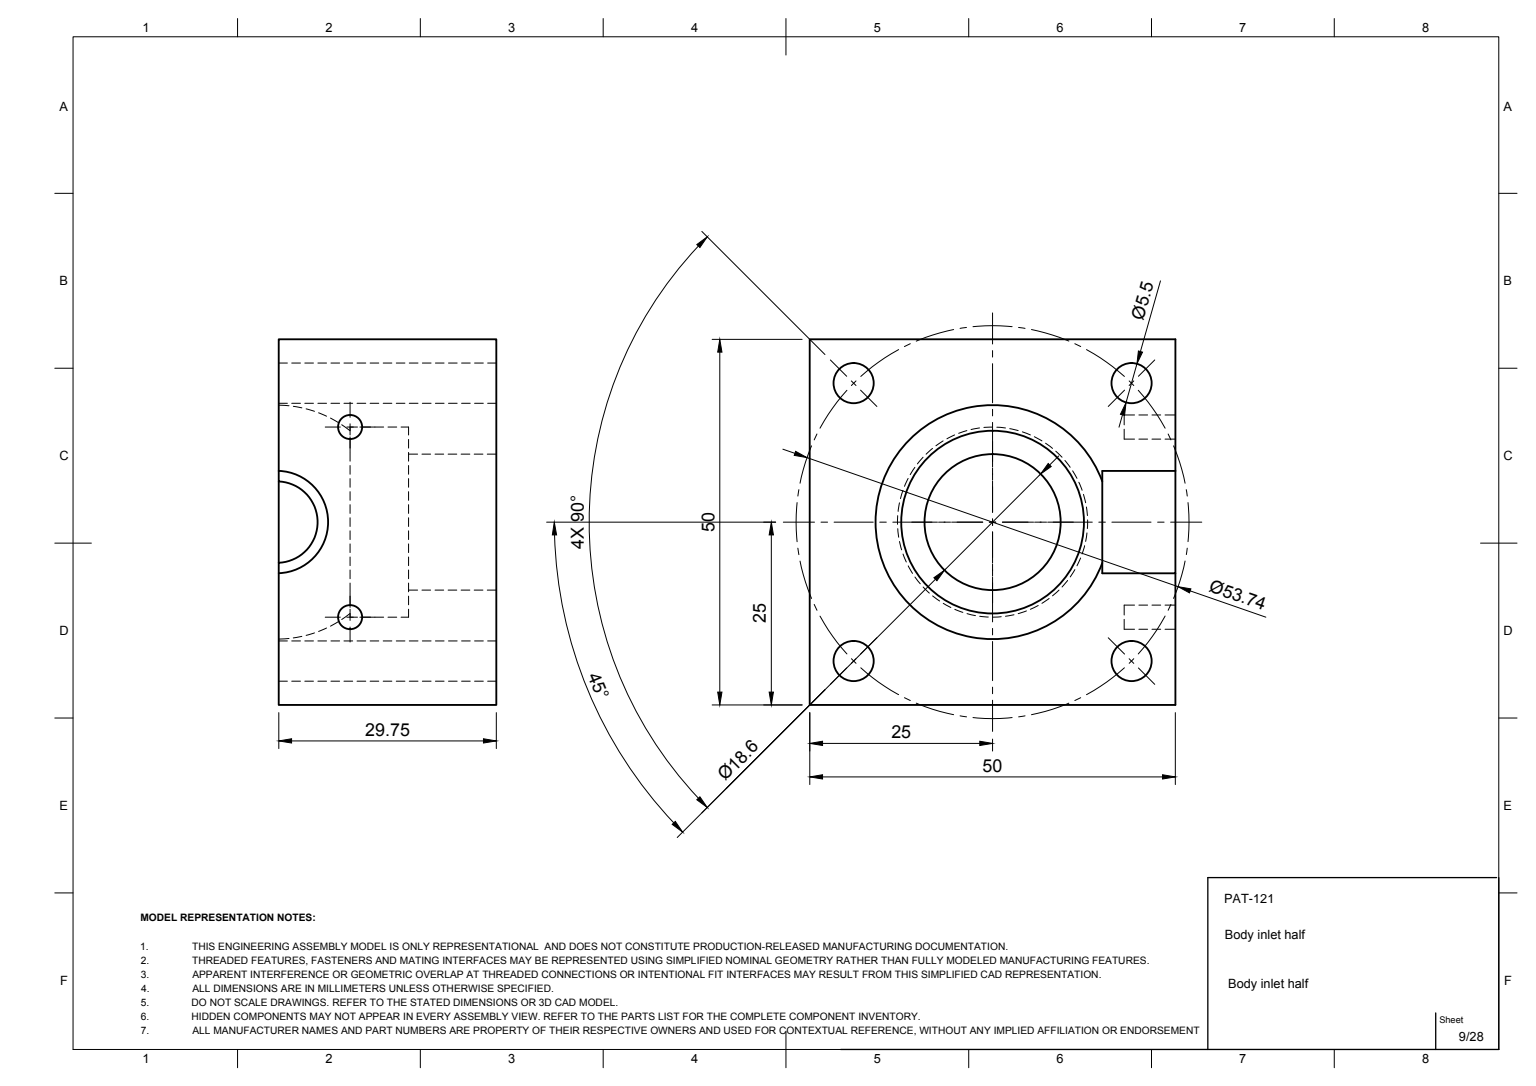
ISO-10303-21;
HEADER;
/* Generated by software containing ST-Developer
 * from STEP Tools, Inc. (www.steptools.com) 
 */

FILE_DESCRIPTION(
/* description */ ('Wall-mounted air drop station'),
/* implementation_level */ '2;1');

FILE_NAME(
/* name */ 'Body inlet half.step',
/* time_stamp */ '2026-10-28T22:16:19-07:00',
/* author */ (''),
/* organization */ (''),
/* preprocessor_version */ 'ST-DEVELOPER v20.2',
/* originating_system */ 'Autodesk Translation Framework v15.17.0.0',
/* authorisation */ '');

FILE_SCHEMA (('AUTOMOTIVE_DESIGN { 1 0 10303 214 3 1 1 }'));
ENDSEC;

DATA;
#10=MECHANICAL_DESIGN_GEOMETRIC_PRESENTATION_REPRESENTATION('',(#349),#10517);
#258=SPHERICAL_SURFACE('',#6417,1.6);
#291=SHAPE_REPRESENTATION_RELATIONSHIP('SRR','None',#10648,#320);
#320=ADVANCED_BREP_SHAPE_REPRESENTATION('',(#378),#10492);
#349=STYLED_ITEM('',(#10853),#378);
#378=MANIFOLD_SOLID_BREP('Body1',#5888);
#435=FACE_BOUND('',#1240,.T.);
#436=FACE_BOUND('',#1241,.T.);
#437=FACE_BOUND('',#1245,.T.);
#438=FACE_BOUND('',#1247,.T.);
#439=FACE_BOUND('',#1249,.T.);
#440=FACE_BOUND('',#1251,.T.);
#441=FACE_BOUND('',#1252,.T.);
#442=FACE_BOUND('',#1253,.T.);
#443=FACE_BOUND('',#1254,.T.);
#444=FACE_BOUND('',#1257,.T.);
#445=FACE_BOUND('',#1258,.T.);
#446=FACE_BOUND('',#1259,.T.);
#447=FACE_BOUND('',#1260,.T.);
#448=FACE_BOUND('',#1261,.T.);
#580=PLANE('',#6385);
#581=PLANE('',#6389);
#582=PLANE('',#6405);
#583=PLANE('',#6407);
#584=PLANE('',#6414);
#585=PLANE('',#6416);
#586=PLANE('',#6419);
#587=PLANE('',#6420);
#588=PLANE('',#6421);
#589=PLANE('',#6422);
#590=PLANE('',#6423);
#838=FACE_OUTER_BOUND('',#1229,.T.);
#839=FACE_OUTER_BOUND('',#1230,.T.);
#840=FACE_OUTER_BOUND('',#1231,.T.);
#841=FACE_OUTER_BOUND('',#1232,.T.);
#842=FACE_OUTER_BOUND('',#1233,.T.);
#843=FACE_OUTER_BOUND('',#1234,.T.);
#844=FACE_OUTER_BOUND('',#1235,.T.);
#845=FACE_OUTER_BOUND('',#1236,.T.);
#846=FACE_OUTER_BOUND('',#1237,.T.);
#847=FACE_OUTER_BOUND('',#1238,.T.);
#848=FACE_OUTER_BOUND('',#1239,.T.);
#849=FACE_OUTER_BOUND('',#1242,.T.);
#850=FACE_OUTER_BOUND('',#1243,.T.);
#851=FACE_OUTER_BOUND('',#1244,.T.);
#852=FACE_OUTER_BOUND('',#1246,.T.);
#853=FACE_OUTER_BOUND('',#1248,.T.);
#854=FACE_OUTER_BOUND('',#1250,.T.);
#855=FACE_OUTER_BOUND('',#1255,.T.);
#856=FACE_OUTER_BOUND('',#1256,.T.);
#857=FACE_OUTER_BOUND('',#1262,.T.);
#858=FACE_OUTER_BOUND('',#1263,.T.);
#1229=EDGE_LOOP('',(#4323,#4324,#4325,#4326));
#1230=EDGE_LOOP('',(#4327));
#1231=EDGE_LOOP('',(#4328,#4329,#4330,#4331));
#1232=EDGE_LOOP('',(#4332));
#1233=EDGE_LOOP('',(#4333,#4334,#4335,#4336));
#1234=EDGE_LOOP('',(#4337,#4338,#4339,#4340));
#1235=EDGE_LOOP('',(#4341,#4342,#4343,#4344));
#1236=EDGE_LOOP('',(#4345,#4346,#4347,#4348));
#1237=EDGE_LOOP('',(#4349,#4350,#4351,#4352));
#1238=EDGE_LOOP('',(#4353,#4354,#4355,#4356));
#1239=EDGE_LOOP('',(#4357,#4358,#4359,#4360,#4361,#4362));
#1240=EDGE_LOOP('',(#4363));
#1241=EDGE_LOOP('',(#4364));
#1242=EDGE_LOOP('',(#4365,#4366,#4367,#4368));
#1243=EDGE_LOOP('',(#4369,#4370,#4371,#4372));
#1244=EDGE_LOOP('',(#4373));
#1245=EDGE_LOOP('',(#4374));
#1246=EDGE_LOOP('',(#4375));
#1247=EDGE_LOOP('',(#4376));
#1248=EDGE_LOOP('',(#4377,#4378));
#1249=EDGE_LOOP('',(#4379));
#1250=EDGE_LOOP('',(#4380,#4381,#4382,#4383,#4384,#4385,#4386,#4387,#4388,
#4389));
#1251=EDGE_LOOP('',(#4390));
#1252=EDGE_LOOP('',(#4391));
#1253=EDGE_LOOP('',(#4392));
#1254=EDGE_LOOP('',(#4393));
#1255=EDGE_LOOP('',(#4394,#4395,#4396,#4397));
#1256=EDGE_LOOP('',(#4398,#4399,#4400,#4401));
#1257=EDGE_LOOP('',(#4402));
#1258=EDGE_LOOP('',(#4403));
#1259=EDGE_LOOP('',(#4404));
#1260=EDGE_LOOP('',(#4405));
#1261=EDGE_LOOP('',(#4406));
#1262=EDGE_LOOP('',(#4407,#4408,#4409,#4410));
#1263=EDGE_LOOP('',(#4411,#4412,#4413,#4414));
#1711=LINE('',#9152,#2175);
#1712=LINE('',#9159,#2176);
#1713=LINE('',#9166,#2177);
#1714=LINE('',#9172,#2178);
#1715=LINE('',#9178,#2179);
#1716=LINE('',#9184,#2180);
#1717=LINE('',#9189,#2181);
#1718=LINE('',#9193,#2182);
#1719=LINE('',#9197,#2183);
#1720=LINE('',#9200,#2184);
#1721=LINE('',#9203,#2185);
#1722=LINE('',#9205,#2186);
#1723=LINE('',#9207,#2187);
#1724=LINE('',#9209,#2188);
#1725=LINE('',#9210,#2189);
#1726=LINE('',#9215,#2190);
#1727=LINE('',#9221,#2191);
#1728=LINE('',#9231,#2192);
#1729=LINE('',#9233,#2193);
#1730=LINE('',#9234,#2194);
#1731=LINE('',#9237,#2195);
#1732=LINE('',#9238,#2196);
#1733=LINE('',#9241,#2197);
#1734=LINE('',#9242,#2198);
#1735=LINE('',#9244,#2199);
#2175=VECTOR('',#7341,0.165);
#2176=VECTOR('',#7350,0.165);
#2177=VECTOR('',#7359,0.275);
#2178=VECTOR('',#7366,0.275);
#2179=VECTOR('',#7373,0.275);
#2180=VECTOR('',#7380,0.275);
#2181=VECTOR('',#7385,1.);
#2182=VECTOR('',#7388,1.);
#2183=VECTOR('',#7393,1.);
#2184=VECTOR('',#7396,1.);
#2185=VECTOR('',#7399,1.);
#2186=VECTOR('',#7400,1.);
#2187=VECTOR('',#7401,1.);
#2188=VECTOR('',#7402,1.);
#2189=VECTOR('',#7403,1.);
#2190=VECTOR('',#7408,0.93);
#2191=VECTOR('',#7415,1.3);
#2192=VECTOR('',#7430,1.);
#2193=VECTOR('',#7431,1.);
#2194=VECTOR('',#7432,1.);
#2195=VECTOR('',#7435,1.);
#2196=VECTOR('',#7436,1.);
#2197=VECTOR('',#7439,1.);
#2198=VECTOR('',#7440,1.);
#2199=VECTOR('',#7443,1.);
#2576=CIRCLE('',#6383,0.165);
#2577=CIRCLE('',#6384,0.165);
#2578=CIRCLE('',#6387,0.165);
#2579=CIRCLE('',#6388,0.165);
#2580=CIRCLE('',#6391,0.275);
#2581=CIRCLE('',#6392,0.275);
#2582=CIRCLE('',#6394,0.275);
#2583=CIRCLE('',#6395,0.275);
#2584=CIRCLE('',#6397,0.275);
#2585=CIRCLE('',#6398,0.275);
#2586=CIRCLE('',#6400,0.275);
#2587=CIRCLE('',#6401,0.275);
#2588=CIRCLE('',#6403,0.7);
#2589=CIRCLE('',#6404,0.7);
#2590=CIRCLE('',#6406,0.556776436283003);
#2591=CIRCLE('',#6409,0.93);
#2592=CIRCLE('',#6410,0.93);
#2593=CIRCLE('',#6412,1.3);
#2594=CIRCLE('',#6413,1.3);
#2595=CIRCLE('',#6415,1.24899959967968);
#2596=CIRCLE('',#6418,1.59980467557762);
#2881=VERTEX_POINT('',#9149);
#2882=VERTEX_POINT('',#9151);
#2883=VERTEX_POINT('',#9156);
#2884=VERTEX_POINT('',#9158);
#2885=VERTEX_POINT('',#9163);
#2886=VERTEX_POINT('',#9165);
#2887=VERTEX_POINT('',#9169);
#2888=VERTEX_POINT('',#9171);
#2889=VERTEX_POINT('',#9175);
#2890=VERTEX_POINT('',#9177);
#2891=VERTEX_POINT('',#9181);
#2892=VERTEX_POINT('',#9183);
#2893=VERTEX_POINT('',#9187);
#2894=VERTEX_POINT('',#9188);
#2895=VERTEX_POINT('',#9190);
#2896=VERTEX_POINT('',#9192);
#2897=VERTEX_POINT('',#9196);
#2898=VERTEX_POINT('',#9198);
#2899=VERTEX_POINT('',#9202);
#2900=VERTEX_POINT('',#9204);
#2901=VERTEX_POINT('',#9206);
#2902=VERTEX_POINT('',#9208);
#2903=VERTEX_POINT('',#9212);
#2904=VERTEX_POINT('',#9214);
#2905=VERTEX_POINT('',#9218);
#2906=VERTEX_POINT('',#9220);
#2907=VERTEX_POINT('',#9224);
#2908=VERTEX_POINT('',#9230);
#2909=VERTEX_POINT('',#9232);
#2910=VERTEX_POINT('',#9236);
#2911=VERTEX_POINT('',#9240);
#3419=EDGE_CURVE('',#2881,#2881,#2576,.T.);
#3420=EDGE_CURVE('',#2881,#2882,#1711,.T.);
#3421=EDGE_CURVE('',#2882,#2882,#2577,.T.);
#3422=EDGE_CURVE('',#2883,#2883,#2578,.T.);
#3423=EDGE_CURVE('',#2883,#2884,#1712,.T.);
#3424=EDGE_CURVE('',#2884,#2884,#2579,.T.);
#3425=EDGE_CURVE('',#2885,#2885,#2580,.T.);
#3426=EDGE_CURVE('',#2885,#2886,#1713,.T.);
#3427=EDGE_CURVE('',#2886,#2886,#2581,.T.);
#3428=EDGE_CURVE('',#2887,#2887,#2582,.T.);
#3429=EDGE_CURVE('',#2887,#2888,#1714,.T.);
#3430=EDGE_CURVE('',#2888,#2888,#2583,.T.);
#3431=EDGE_CURVE('',#2889,#2889,#2584,.T.);
#3432=EDGE_CURVE('',#2889,#2890,#1715,.T.);
#3433=EDGE_CURVE('',#2890,#2890,#2585,.T.);
#3434=EDGE_CURVE('',#2891,#2891,#2586,.T.);
#3435=EDGE_CURVE('',#2891,#2892,#1716,.T.);
#3436=EDGE_CURVE('',#2892,#2892,#2587,.T.);
#3437=EDGE_CURVE('',#2893,#2894,#1717,.T.);
#3438=EDGE_CURVE('',#2895,#2893,#2588,.T.);
#3439=EDGE_CURVE('',#2896,#2895,#1718,.T.);
#3440=EDGE_CURVE('',#2894,#2896,#2589,.T.);
#3441=EDGE_CURVE('',#2897,#2893,#1719,.T.);
#3442=EDGE_CURVE('',#2898,#2897,#2590,.T.);
#3443=EDGE_CURVE('',#2895,#2898,#1720,.T.);
#3444=EDGE_CURVE('',#2896,#2899,#1721,.T.);
#3445=EDGE_CURVE('',#2899,#2900,#1722,.T.);
#3446=EDGE_CURVE('',#2900,#2901,#1723,.T.);
#3447=EDGE_CURVE('',#2901,#2902,#1724,.T.);
#3448=EDGE_CURVE('',#2902,#2894,#1725,.T.);
#3449=EDGE_CURVE('',#2903,#2903,#2591,.T.);
#3450=EDGE_CURVE('',#2903,#2904,#1726,.T.);
#3451=EDGE_CURVE('',#2904,#2904,#2592,.T.);
#3452=EDGE_CURVE('',#2905,#2905,#2593,.T.);
#3453=EDGE_CURVE('',#2905,#2906,#1727,.T.);
#3454=EDGE_CURVE('',#2906,#2906,#2594,.T.);
#3455=EDGE_CURVE('',#2907,#2907,#2595,.T.);
#3456=EDGE_CURVE('',#2898,#2897,#2596,.T.);
#3457=EDGE_CURVE('',#2908,#2902,#1728,.T.);
#3458=EDGE_CURVE('',#2908,#2909,#1729,.T.);
#3459=EDGE_CURVE('',#2909,#2899,#1730,.T.);
#3460=EDGE_CURVE('',#2910,#2908,#1731,.T.);
#3461=EDGE_CURVE('',#2910,#2901,#1732,.T.);
#3462=EDGE_CURVE('',#2911,#2910,#1733,.T.);
#3463=EDGE_CURVE('',#2911,#2900,#1734,.T.);
#3464=EDGE_CURVE('',#2909,#2911,#1735,.T.);
#4323=ORIENTED_EDGE('',*,*,#3419,.F.);
#4324=ORIENTED_EDGE('',*,*,#3420,.T.);
#4325=ORIENTED_EDGE('',*,*,#3421,.F.);
#4326=ORIENTED_EDGE('',*,*,#3420,.F.);
#4327=ORIENTED_EDGE('',*,*,#3419,.T.);
#4328=ORIENTED_EDGE('',*,*,#3422,.F.);
#4329=ORIENTED_EDGE('',*,*,#3423,.T.);
#4330=ORIENTED_EDGE('',*,*,#3424,.F.);
#4331=ORIENTED_EDGE('',*,*,#3423,.F.);
#4332=ORIENTED_EDGE('',*,*,#3422,.T.);
#4333=ORIENTED_EDGE('',*,*,#3425,.F.);
#4334=ORIENTED_EDGE('',*,*,#3426,.T.);
#4335=ORIENTED_EDGE('',*,*,#3427,.F.);
#4336=ORIENTED_EDGE('',*,*,#3426,.F.);
#4337=ORIENTED_EDGE('',*,*,#3428,.F.);
#4338=ORIENTED_EDGE('',*,*,#3429,.T.);
#4339=ORIENTED_EDGE('',*,*,#3430,.F.);
#4340=ORIENTED_EDGE('',*,*,#3429,.F.);
#4341=ORIENTED_EDGE('',*,*,#3431,.F.);
#4342=ORIENTED_EDGE('',*,*,#3432,.T.);
#4343=ORIENTED_EDGE('',*,*,#3433,.F.);
#4344=ORIENTED_EDGE('',*,*,#3432,.F.);
#4345=ORIENTED_EDGE('',*,*,#3434,.F.);
#4346=ORIENTED_EDGE('',*,*,#3435,.T.);
#4347=ORIENTED_EDGE('',*,*,#3436,.F.);
#4348=ORIENTED_EDGE('',*,*,#3435,.F.);
#4349=ORIENTED_EDGE('',*,*,#3437,.F.);
#4350=ORIENTED_EDGE('',*,*,#3438,.F.);
#4351=ORIENTED_EDGE('',*,*,#3439,.F.);
#4352=ORIENTED_EDGE('',*,*,#3440,.F.);
#4353=ORIENTED_EDGE('',*,*,#3441,.F.);
#4354=ORIENTED_EDGE('',*,*,#3442,.F.);
#4355=ORIENTED_EDGE('',*,*,#3443,.F.);
#4356=ORIENTED_EDGE('',*,*,#3438,.T.);
#4357=ORIENTED_EDGE('',*,*,#3440,.T.);
#4358=ORIENTED_EDGE('',*,*,#3444,.T.);
#4359=ORIENTED_EDGE('',*,*,#3445,.T.);
#4360=ORIENTED_EDGE('',*,*,#3446,.T.);
#4361=ORIENTED_EDGE('',*,*,#3447,.T.);
#4362=ORIENTED_EDGE('',*,*,#3448,.T.);
#4363=ORIENTED_EDGE('',*,*,#3421,.T.);
#4364=ORIENTED_EDGE('',*,*,#3424,.T.);
#4365=ORIENTED_EDGE('',*,*,#3449,.F.);
#4366=ORIENTED_EDGE('',*,*,#3450,.T.);
#4367=ORIENTED_EDGE('',*,*,#3451,.F.);
#4368=ORIENTED_EDGE('',*,*,#3450,.F.);
#4369=ORIENTED_EDGE('',*,*,#3452,.F.);
#4370=ORIENTED_EDGE('',*,*,#3453,.T.);
#4371=ORIENTED_EDGE('',*,*,#3454,.T.);
#4372=ORIENTED_EDGE('',*,*,#3453,.F.);
#4373=ORIENTED_EDGE('',*,*,#3454,.F.);
#4374=ORIENTED_EDGE('',*,*,#3455,.F.);
#4375=ORIENTED_EDGE('',*,*,#3452,.T.);
#4376=ORIENTED_EDGE('',*,*,#3451,.T.);
#4377=ORIENTED_EDGE('',*,*,#3442,.T.);
#4378=ORIENTED_EDGE('',*,*,#3456,.F.);
#4379=ORIENTED_EDGE('',*,*,#3455,.T.);
#4380=ORIENTED_EDGE('',*,*,#3437,.T.);
#4381=ORIENTED_EDGE('',*,*,#3448,.F.);
#4382=ORIENTED_EDGE('',*,*,#3457,.F.);
#4383=ORIENTED_EDGE('',*,*,#3458,.T.);
#4384=ORIENTED_EDGE('',*,*,#3459,.T.);
#4385=ORIENTED_EDGE('',*,*,#3444,.F.);
#4386=ORIENTED_EDGE('',*,*,#3439,.T.);
#4387=ORIENTED_EDGE('',*,*,#3443,.T.);
#4388=ORIENTED_EDGE('',*,*,#3456,.T.);
#4389=ORIENTED_EDGE('',*,*,#3441,.T.);
#4390=ORIENTED_EDGE('',*,*,#3427,.T.);
#4391=ORIENTED_EDGE('',*,*,#3430,.T.);
#4392=ORIENTED_EDGE('',*,*,#3433,.T.);
#4393=ORIENTED_EDGE('',*,*,#3436,.T.);
#4394=ORIENTED_EDGE('',*,*,#3460,.T.);
#4395=ORIENTED_EDGE('',*,*,#3457,.T.);
#4396=ORIENTED_EDGE('',*,*,#3447,.F.);
#4397=ORIENTED_EDGE('',*,*,#3461,.F.);
#4398=ORIENTED_EDGE('',*,*,#3462,.T.);
#4399=ORIENTED_EDGE('',*,*,#3461,.T.);
#4400=ORIENTED_EDGE('',*,*,#3446,.F.);
#4401=ORIENTED_EDGE('',*,*,#3463,.F.);
#4402=ORIENTED_EDGE('',*,*,#3449,.T.);
#4403=ORIENTED_EDGE('',*,*,#3434,.T.);
#4404=ORIENTED_EDGE('',*,*,#3431,.T.);
#4405=ORIENTED_EDGE('',*,*,#3428,.T.);
#4406=ORIENTED_EDGE('',*,*,#3425,.T.);
#4407=ORIENTED_EDGE('',*,*,#3464,.T.);
#4408=ORIENTED_EDGE('',*,*,#3463,.T.);
#4409=ORIENTED_EDGE('',*,*,#3445,.F.);
#4410=ORIENTED_EDGE('',*,*,#3459,.F.);
#4411=ORIENTED_EDGE('',*,*,#3464,.F.);
#4412=ORIENTED_EDGE('',*,*,#3458,.F.);
#4413=ORIENTED_EDGE('',*,*,#3460,.F.);
#4414=ORIENTED_EDGE('',*,*,#3462,.F.);
#5457=CYLINDRICAL_SURFACE('',#6382,0.165);
#5458=CYLINDRICAL_SURFACE('',#6386,0.165);
#5459=CYLINDRICAL_SURFACE('',#6390,0.275);
#5460=CYLINDRICAL_SURFACE('',#6393,0.275);
#5461=CYLINDRICAL_SURFACE('',#6396,0.275);
#5462=CYLINDRICAL_SURFACE('',#6399,0.275);
#5463=CYLINDRICAL_SURFACE('',#6402,0.7);
#5464=CYLINDRICAL_SURFACE('',#6408,0.93);
#5465=CYLINDRICAL_SURFACE('',#6411,1.3);
#5611=ADVANCED_FACE('',(#838),#5457,.F.);
#5612=ADVANCED_FACE('',(#839),#580,.T.);
#5613=ADVANCED_FACE('',(#840),#5458,.F.);
#5614=ADVANCED_FACE('',(#841),#581,.T.);
#5615=ADVANCED_FACE('',(#842),#5459,.F.);
#5616=ADVANCED_FACE('',(#843),#5460,.F.);
#5617=ADVANCED_FACE('',(#844),#5461,.F.);
#5618=ADVANCED_FACE('',(#845),#5462,.F.);
#5619=ADVANCED_FACE('',(#846),#5463,.F.);
#5620=ADVANCED_FACE('',(#847),#582,.T.);
#5621=ADVANCED_FACE('',(#848,#435,#436),#583,.T.);
#5622=ADVANCED_FACE('',(#849),#5464,.F.);
#5623=ADVANCED_FACE('',(#850),#5465,.F.);
#5624=ADVANCED_FACE('',(#851,#437),#584,.F.);
#5625=ADVANCED_FACE('',(#852,#438),#585,.T.);
#5626=ADVANCED_FACE('',(#853,#439),#258,.F.);
#5627=ADVANCED_FACE('',(#854,#440,#441,#442,#443),#586,.T.);
#5628=ADVANCED_FACE('',(#855),#587,.T.);
#5629=ADVANCED_FACE('',(#856,#444,#445,#446,#447,#448),#588,.T.);
#5630=ADVANCED_FACE('',(#857),#589,.T.);
#5631=ADVANCED_FACE('',(#858),#590,.F.);
#5888=CLOSED_SHELL('',(#5611,#5612,#5613,#5614,#5615,#5616,#5617,#5618,
#5619,#5620,#5621,#5622,#5623,#5624,#5625,#5626,#5627,#5628,#5629,#5630,
#5631));
#6381=AXIS2_PLACEMENT_3D('',#9147,#7335,#7336);
#6382=AXIS2_PLACEMENT_3D('',#9148,#7337,#7338);
#6383=AXIS2_PLACEMENT_3D('',#9150,#7339,#7340);
#6384=AXIS2_PLACEMENT_3D('',#9153,#7342,#7343);
#6385=AXIS2_PLACEMENT_3D('',#9154,#7344,#7345);
#6386=AXIS2_PLACEMENT_3D('',#9155,#7346,#7347);
#6387=AXIS2_PLACEMENT_3D('',#9157,#7348,#7349);
#6388=AXIS2_PLACEMENT_3D('',#9160,#7351,#7352);
#6389=AXIS2_PLACEMENT_3D('',#9161,#7353,#7354);
#6390=AXIS2_PLACEMENT_3D('',#9162,#7355,#7356);
#6391=AXIS2_PLACEMENT_3D('',#9164,#7357,#7358);
#6392=AXIS2_PLACEMENT_3D('',#9167,#7360,#7361);
#6393=AXIS2_PLACEMENT_3D('',#9168,#7362,#7363);
#6394=AXIS2_PLACEMENT_3D('',#9170,#7364,#7365);
#6395=AXIS2_PLACEMENT_3D('',#9173,#7367,#7368);
#6396=AXIS2_PLACEMENT_3D('',#9174,#7369,#7370);
#6397=AXIS2_PLACEMENT_3D('',#9176,#7371,#7372);
#6398=AXIS2_PLACEMENT_3D('',#9179,#7374,#7375);
#6399=AXIS2_PLACEMENT_3D('',#9180,#7376,#7377);
#6400=AXIS2_PLACEMENT_3D('',#9182,#7378,#7379);
#6401=AXIS2_PLACEMENT_3D('',#9185,#7381,#7382);
#6402=AXIS2_PLACEMENT_3D('',#9186,#7383,#7384);
#6403=AXIS2_PLACEMENT_3D('',#9191,#7386,#7387);
#6404=AXIS2_PLACEMENT_3D('',#9194,#7389,#7390);
#6405=AXIS2_PLACEMENT_3D('',#9195,#7391,#7392);
#6406=AXIS2_PLACEMENT_3D('',#9199,#7394,#7395);
#6407=AXIS2_PLACEMENT_3D('',#9201,#7397,#7398);
#6408=AXIS2_PLACEMENT_3D('',#9211,#7404,#7405);
#6409=AXIS2_PLACEMENT_3D('',#9213,#7406,#7407);
#6410=AXIS2_PLACEMENT_3D('',#9216,#7409,#7410);
#6411=AXIS2_PLACEMENT_3D('',#9217,#7411,#7412);
#6412=AXIS2_PLACEMENT_3D('',#9219,#7413,#7414);
#6413=AXIS2_PLACEMENT_3D('',#9222,#7416,#7417);
#6414=AXIS2_PLACEMENT_3D('',#9223,#7418,#7419);
#6415=AXIS2_PLACEMENT_3D('',#9225,#7420,#7421);
#6416=AXIS2_PLACEMENT_3D('',#9226,#7422,#7423);
#6417=AXIS2_PLACEMENT_3D('',#9227,#7424,#7425);
#6418=AXIS2_PLACEMENT_3D('',#9228,#7426,#7427);
#6419=AXIS2_PLACEMENT_3D('',#9229,#7428,#7429);
#6420=AXIS2_PLACEMENT_3D('',#9235,#7433,#7434);
#6421=AXIS2_PLACEMENT_3D('',#9239,#7437,#7438);
#6422=AXIS2_PLACEMENT_3D('',#9243,#7441,#7442);
#6423=AXIS2_PLACEMENT_3D('',#9245,#7444,#7445);
#7335=DIRECTION('axis',(0.,0.,1.));
#7336=DIRECTION('refdir',(1.,0.,0.));
#7337=DIRECTION('center_axis',(0.,0.,1.));
#7338=DIRECTION('ref_axis',(1.,0.,0.));
#7339=DIRECTION('center_axis',(0.,0.,1.));
#7340=DIRECTION('ref_axis',(1.,0.,0.));
#7341=DIRECTION('',(0.,0.,1.));
#7342=DIRECTION('center_axis',(0.,0.,-1.));
#7343=DIRECTION('ref_axis',(1.,0.,0.));
#7344=DIRECTION('center_axis',(0.,0.,1.));
#7345=DIRECTION('ref_axis',(1.,0.,0.));
#7346=DIRECTION('center_axis',(0.,0.,1.));
#7347=DIRECTION('ref_axis',(1.,0.,0.));
#7348=DIRECTION('center_axis',(0.,0.,1.));
#7349=DIRECTION('ref_axis',(1.,0.,0.));
#7350=DIRECTION('',(0.,0.,1.));
#7351=DIRECTION('center_axis',(0.,0.,-1.));
#7352=DIRECTION('ref_axis',(1.,0.,0.));
#7353=DIRECTION('center_axis',(0.,0.,1.));
#7354=DIRECTION('ref_axis',(1.,0.,0.));
#7355=DIRECTION('center_axis',(0.,1.,0.));
#7356=DIRECTION('ref_axis',(1.,0.,0.));
#7357=DIRECTION('center_axis',(0.,1.,0.));
#7358=DIRECTION('ref_axis',(1.,0.,0.));
#7359=DIRECTION('',(0.,1.,0.));
#7360=DIRECTION('center_axis',(0.,-1.,0.));
#7361=DIRECTION('ref_axis',(1.,0.,0.));
#7362=DIRECTION('center_axis',(0.,1.,0.));
#7363=DIRECTION('ref_axis',(1.,0.,0.));
#7364=DIRECTION('center_axis',(0.,1.,0.));
#7365=DIRECTION('ref_axis',(1.,0.,0.));
#7366=DIRECTION('',(0.,1.,0.));
#7367=DIRECTION('center_axis',(0.,-1.,0.));
#7368=DIRECTION('ref_axis',(1.,0.,0.));
#7369=DIRECTION('center_axis',(0.,1.,0.));
#7370=DIRECTION('ref_axis',(1.,0.,0.));
#7371=DIRECTION('center_axis',(0.,1.,0.));
#7372=DIRECTION('ref_axis',(1.,0.,0.));
#7373=DIRECTION('',(0.,1.,0.));
#7374=DIRECTION('center_axis',(0.,-1.,0.));
#7375=DIRECTION('ref_axis',(1.,0.,0.));
#7376=DIRECTION('center_axis',(0.,1.,0.));
#7377=DIRECTION('ref_axis',(1.,0.,0.));
#7378=DIRECTION('center_axis',(0.,1.,0.));
#7379=DIRECTION('ref_axis',(1.,0.,0.));
#7380=DIRECTION('',(0.,1.,0.));
#7381=DIRECTION('center_axis',(0.,-1.,0.));
#7382=DIRECTION('ref_axis',(1.,0.,0.));
#7383=DIRECTION('center_axis',(0.,0.,1.));
#7384=DIRECTION('ref_axis',(1.,0.,0.));
#7385=DIRECTION('',(0.,0.,1.));
#7386=DIRECTION('center_axis',(0.,0.,1.));
#7387=DIRECTION('ref_axis',(1.,0.,0.));
#7388=DIRECTION('',(0.,0.,-1.));
#7389=DIRECTION('center_axis',(0.,0.,-1.));
#7390=DIRECTION('ref_axis',(1.,0.,0.));
#7391=DIRECTION('center_axis',(0.,0.,1.));
#7392=DIRECTION('ref_axis',(1.,0.,0.));
#7393=DIRECTION('',(1.,0.,0.));
#7394=DIRECTION('center_axis',(0.,0.,1.));
#7395=DIRECTION('ref_axis',(0.,-1.,0.));
#7396=DIRECTION('',(1.,0.,0.));
#7397=DIRECTION('center_axis',(0.,0.,1.));
#7398=DIRECTION('ref_axis',(1.,0.,0.));
#7399=DIRECTION('',(-1.,0.,0.));
#7400=DIRECTION('',(0.,-1.,0.));
#7401=DIRECTION('',(1.,0.,0.));
#7402=DIRECTION('',(0.,1.,0.));
#7403=DIRECTION('',(-1.,0.,0.));
#7404=DIRECTION('center_axis',(0.,1.,0.));
#7405=DIRECTION('ref_axis',(1.,0.,0.));
#7406=DIRECTION('center_axis',(0.,1.,0.));
#7407=DIRECTION('ref_axis',(1.,0.,0.));
#7408=DIRECTION('',(0.,1.,0.));
#7409=DIRECTION('center_axis',(0.,-1.,0.));
#7410=DIRECTION('ref_axis',(1.,0.,0.));
#7411=DIRECTION('center_axis',(0.,1.,0.));
#7412=DIRECTION('ref_axis',(1.,0.,0.));
#7413=DIRECTION('center_axis',(0.,1.,0.));
#7414=DIRECTION('ref_axis',(1.,0.,0.));
#7415=DIRECTION('',(0.,1.,0.));
#7416=DIRECTION('center_axis',(0.,1.,0.));
#7417=DIRECTION('ref_axis',(1.,0.,0.));
#7418=DIRECTION('center_axis',(0.,1.,0.));
#7419=DIRECTION('ref_axis',(1.,0.,0.));
#7420=DIRECTION('center_axis',(0.,-1.,0.));
#7421=DIRECTION('ref_axis',(0.,0.,-1.));
#7422=DIRECTION('center_axis',(0.,1.,0.));
#7423=DIRECTION('ref_axis',(1.,0.,0.));
#7424=DIRECTION('center_axis',(6.12323399573677E-17,0.,1.));
#7425=DIRECTION('ref_axis',(1.,0.,0.));
#7426=DIRECTION('center_axis',(0.,-1.,0.));
#7427=DIRECTION('ref_axis',(0.,0.,-1.));
#7428=DIRECTION('center_axis',(0.,1.,0.));
#7429=DIRECTION('ref_axis',(-1.,0.,0.));
#7430=DIRECTION('',(0.,0.,1.));
#7431=DIRECTION('',(-1.,0.,0.));
#7432=DIRECTION('',(0.,0.,1.));
#7433=DIRECTION('center_axis',(1.,0.,0.));
#7434=DIRECTION('ref_axis',(0.,1.,0.));
#7435=DIRECTION('',(0.,1.,0.));
#7436=DIRECTION('',(0.,0.,1.));
#7437=DIRECTION('center_axis',(0.,-1.,0.));
#7438=DIRECTION('ref_axis',(1.,0.,0.));
#7439=DIRECTION('',(1.,0.,0.));
#7440=DIRECTION('',(0.,0.,1.));
#7441=DIRECTION('center_axis',(-1.,0.,0.));
#7442=DIRECTION('ref_axis',(0.,-1.,0.));
#7443=DIRECTION('',(0.,-1.,0.));
#7444=DIRECTION('center_axis',(0.,0.,1.));
#7445=DIRECTION('ref_axis',(1.,0.,0.));
#9147=CARTESIAN_POINT('',(0.,0.,0.));
#9148=CARTESIAN_POINT('Origin',(-1.3,-1.,6.8));
#9149=CARTESIAN_POINT('',(-1.465,-1.,6.8));
#9150=CARTESIAN_POINT('Origin',(-1.3,-1.,6.8));
#9151=CARTESIAN_POINT('',(-1.465,-1.,7.5));
#9152=CARTESIAN_POINT('',(-1.465,-1.,6.8));
#9153=CARTESIAN_POINT('Origin',(-1.3,-1.,7.5));
#9154=CARTESIAN_POINT('Origin',(-1.3,-1.,6.8));
#9155=CARTESIAN_POINT('Origin',(1.3,-1.,6.8));
#9156=CARTESIAN_POINT('',(1.135,-1.,6.8));
#9157=CARTESIAN_POINT('Origin',(1.3,-1.,6.8));
#9158=CARTESIAN_POINT('',(1.135,-1.,7.5));
#9159=CARTESIAN_POINT('',(1.135,-1.,6.8));
#9160=CARTESIAN_POINT('Origin',(1.3,-1.,7.5));
#9161=CARTESIAN_POINT('Origin',(1.3,-1.,6.8));
#9162=CARTESIAN_POINT('Origin',(1.9,-3.1,3.1));
#9163=CARTESIAN_POINT('',(1.625,-3.,3.1));
#9164=CARTESIAN_POINT('Origin',(1.9,-3.,3.1));
#9165=CARTESIAN_POINT('',(1.625,-0.0249999999999999,3.1));
#9166=CARTESIAN_POINT('',(1.625,-3.1,3.1));
#9167=CARTESIAN_POINT('Origin',(1.9,-0.0249999999999999,3.1));
#9168=CARTESIAN_POINT('Origin',(-1.9,-3.1,6.9));
#9169=CARTESIAN_POINT('',(-2.175,-3.,6.9));
#9170=CARTESIAN_POINT('Origin',(-1.9,-3.,6.9));
#9171=CARTESIAN_POINT('',(-2.175,-0.0249999999999999,6.9));
#9172=CARTESIAN_POINT('',(-2.175,-3.1,6.9));
#9173=CARTESIAN_POINT('Origin',(-1.9,-0.0249999999999999,6.9));
#9174=CARTESIAN_POINT('Origin',(-1.9,-3.1,3.1));
#9175=CARTESIAN_POINT('',(-2.175,-3.,3.1));
#9176=CARTESIAN_POINT('Origin',(-1.9,-3.,3.1));
#9177=CARTESIAN_POINT('',(-2.175,-0.0249999999999999,3.1));
#9178=CARTESIAN_POINT('',(-2.175,-3.1,3.1));
#9179=CARTESIAN_POINT('Origin',(-1.9,-0.0249999999999999,3.1));
#9180=CARTESIAN_POINT('Origin',(1.9,-3.1,6.9));
#9181=CARTESIAN_POINT('',(1.625,-3.,6.9));
#9182=CARTESIAN_POINT('Origin',(1.9,-3.,6.9));
#9183=CARTESIAN_POINT('',(1.625,-0.0249999999999999,6.9));
#9184=CARTESIAN_POINT('',(1.625,-3.1,6.9));
#9185=CARTESIAN_POINT('Origin',(1.9,-0.0249999999999999,6.9));
#9186=CARTESIAN_POINT('Origin',(0.,0.,6.5));
#9187=CARTESIAN_POINT('',(0.699553428981661,-0.025,6.5));
#9188=CARTESIAN_POINT('',(0.699553428981661,-0.025,7.5));
#9189=CARTESIAN_POINT('',(0.699553428981661,-0.025,6.5));
#9190=CARTESIAN_POINT('',(-0.699553428981661,-0.025,6.5));
#9191=CARTESIAN_POINT('Origin',(0.,0.,6.5));
#9192=CARTESIAN_POINT('',(-0.699553428981661,-0.025,7.5));
#9193=CARTESIAN_POINT('',(-0.699553428981661,-0.025,6.5));
#9194=CARTESIAN_POINT('Origin',(0.,0.,7.5));
#9195=CARTESIAN_POINT('Origin',(0.,0.,6.5));
#9196=CARTESIAN_POINT('',(0.556214886532175,-0.025,6.5));
#9197=CARTESIAN_POINT('',(1.25,-0.025,6.5));
#9198=CARTESIAN_POINT('',(-0.556214886532175,-0.025,6.5));
#9199=CARTESIAN_POINT('Origin',(0.,0.,6.5));
#9200=CARTESIAN_POINT('',(1.25,-0.025,6.5));
#9201=CARTESIAN_POINT('Origin',(0.,-1.5125,7.5));
#9202=CARTESIAN_POINT('',(-2.5,-0.025,7.5));
#9203=CARTESIAN_POINT('',(2.5,-0.025,7.5));
#9204=CARTESIAN_POINT('',(-2.5,-3.,7.5));
#9205=CARTESIAN_POINT('',(-2.5,-0.025,7.5));
#9206=CARTESIAN_POINT('',(2.5,-3.,7.5));
#9207=CARTESIAN_POINT('',(-2.5,-3.,7.5));
#9208=CARTESIAN_POINT('',(2.5,-0.025,7.5));
#9209=CARTESIAN_POINT('',(2.5,-3.,7.5));
#9210=CARTESIAN_POINT('',(2.5,-0.025,7.5));
#9211=CARTESIAN_POINT('Origin',(0.,-3.1,5.));
#9212=CARTESIAN_POINT('',(-0.93,-3.,5.));
#9213=CARTESIAN_POINT('Origin',(0.,-3.,5.));
#9214=CARTESIAN_POINT('',(-0.93,-1.8,5.));
#9215=CARTESIAN_POINT('',(-0.93,-3.1,5.));
#9216=CARTESIAN_POINT('Origin',(0.,-1.8,5.));
#9217=CARTESIAN_POINT('Origin',(0.,-1.8,5.));
#9218=CARTESIAN_POINT('',(-1.3,-1.8,5.));
#9219=CARTESIAN_POINT('Origin',(0.,-1.8,5.));
#9220=CARTESIAN_POINT('',(-1.3,-1.,5.));
#9221=CARTESIAN_POINT('',(-1.3,-1.8,5.));
#9222=CARTESIAN_POINT('Origin',(0.,-1.,5.));
#9223=CARTESIAN_POINT('Origin',(0.,-1.,5.));
#9224=CARTESIAN_POINT('',(-1.52958336188405E-16,-1.,6.24899959967968));
#9225=CARTESIAN_POINT('Origin',(0.,-1.,5.));
#9226=CARTESIAN_POINT('Origin',(0.,-1.8,5.));
#9227=CARTESIAN_POINT('Origin',(0.,0.,5.));
#9228=CARTESIAN_POINT('Origin',(0.,-0.025,5.));
#9229=CARTESIAN_POINT('Origin',(2.5,-0.025,2.5));
#9230=CARTESIAN_POINT('',(2.5,-0.025,2.5));
#9231=CARTESIAN_POINT('',(2.5,-0.025,2.5));
#9232=CARTESIAN_POINT('',(-2.5,-0.025,2.5));
#9233=CARTESIAN_POINT('',(2.5,-0.025,2.5));
#9234=CARTESIAN_POINT('',(-2.5,-0.025,2.5));
#9235=CARTESIAN_POINT('Origin',(2.5,-3.,2.5));
#9236=CARTESIAN_POINT('',(2.5,-3.,2.5));
#9237=CARTESIAN_POINT('',(2.5,-3.,2.5));
#9238=CARTESIAN_POINT('',(2.5,-3.,2.5));
#9239=CARTESIAN_POINT('Origin',(-2.5,-3.,2.5));
#9240=CARTESIAN_POINT('',(-2.5,-3.,2.5));
#9241=CARTESIAN_POINT('',(-2.5,-3.,2.5));
#9242=CARTESIAN_POINT('',(-2.5,-3.,2.5));
#9243=CARTESIAN_POINT('Origin',(-2.5,-0.025,2.5));
#9244=CARTESIAN_POINT('',(-2.5,-0.025,2.5));
#9245=CARTESIAN_POINT('Origin',(0.,-1.5125,2.5));
#10459=UNCERTAINTY_MEASURE_WITH_UNIT(LENGTH_MEASURE(0.001),#10518,
'DISTANCE_ACCURACY_VALUE',
'Maximum model space distance between geometric entities at asserted c
onnectivities');
#10484=UNCERTAINTY_MEASURE_WITH_UNIT(LENGTH_MEASURE(0.001),#10518,
'DISTANCE_ACCURACY_VALUE',
'Maximum model space distance between geometric entities at asserted c
onnectivities');
#10492=(
GEOMETRIC_REPRESENTATION_CONTEXT(3)
GLOBAL_UNCERTAINTY_ASSIGNED_CONTEXT((#10459))
GLOBAL_UNIT_ASSIGNED_CONTEXT((#10518,#10520,#10521))
REPRESENTATION_CONTEXT('','3D')
);
#10517=(
GEOMETRIC_REPRESENTATION_CONTEXT(3)
GLOBAL_UNCERTAINTY_ASSIGNED_CONTEXT((#10484))
GLOBAL_UNIT_ASSIGNED_CONTEXT((#10518,#10520,#10521))
REPRESENTATION_CONTEXT('','3D')
);
#10518=(
LENGTH_UNIT()
NAMED_UNIT(*)
SI_UNIT(.CENTI.,.METRE.)
);
#10520=(
NAMED_UNIT(*)
PLANE_ANGLE_UNIT()
SI_UNIT($,.RADIAN.)
);
#10521=(
NAMED_UNIT(*)
SI_UNIT($,.STERADIAN.)
SOLID_ANGLE_UNIT()
);
#10529=SHAPE_DEFINITION_REPRESENTATION(#10561,#10648);
#10561=PRODUCT_DEFINITION_SHAPE('',$,#10681);
#10648=SHAPE_REPRESENTATION('',(#6381),#10492);
#10673=PRODUCT_DEFINITION_CONTEXT('part definition',#10771,'design');
#10681=PRODUCT_DEFINITION('Body inlet half','Body inlet half',#10713,#10673);
#10713=PRODUCT_DEFINITION_FORMATION('',$,#10780);
#10771=APPLICATION_CONTEXT(
'Core Data for Automotive Mechanical Design Process');
#10772=PRODUCT_CONTEXT('part definition',#10771,'mechanical');
#10780=PRODUCT('Body inlet half','Body inlet half','Body inlet half',(#10772));
#10847=COLOUR_RGB('Dark Blue',0.08,0.2,0.34);
#10848=FILL_AREA_STYLE_COLOUR('',#10847);
#10849=FILL_AREA_STYLE('',(#10848));
#10850=SURFACE_STYLE_FILL_AREA(#10849);
#10851=SURFACE_SIDE_STYLE('',(#10850));
#10852=SURFACE_STYLE_USAGE(.BOTH.,#10851);
#10853=PRESENTATION_STYLE_ASSIGNMENT((#10852));
ENDSEC;
END-ISO-10303-21;
